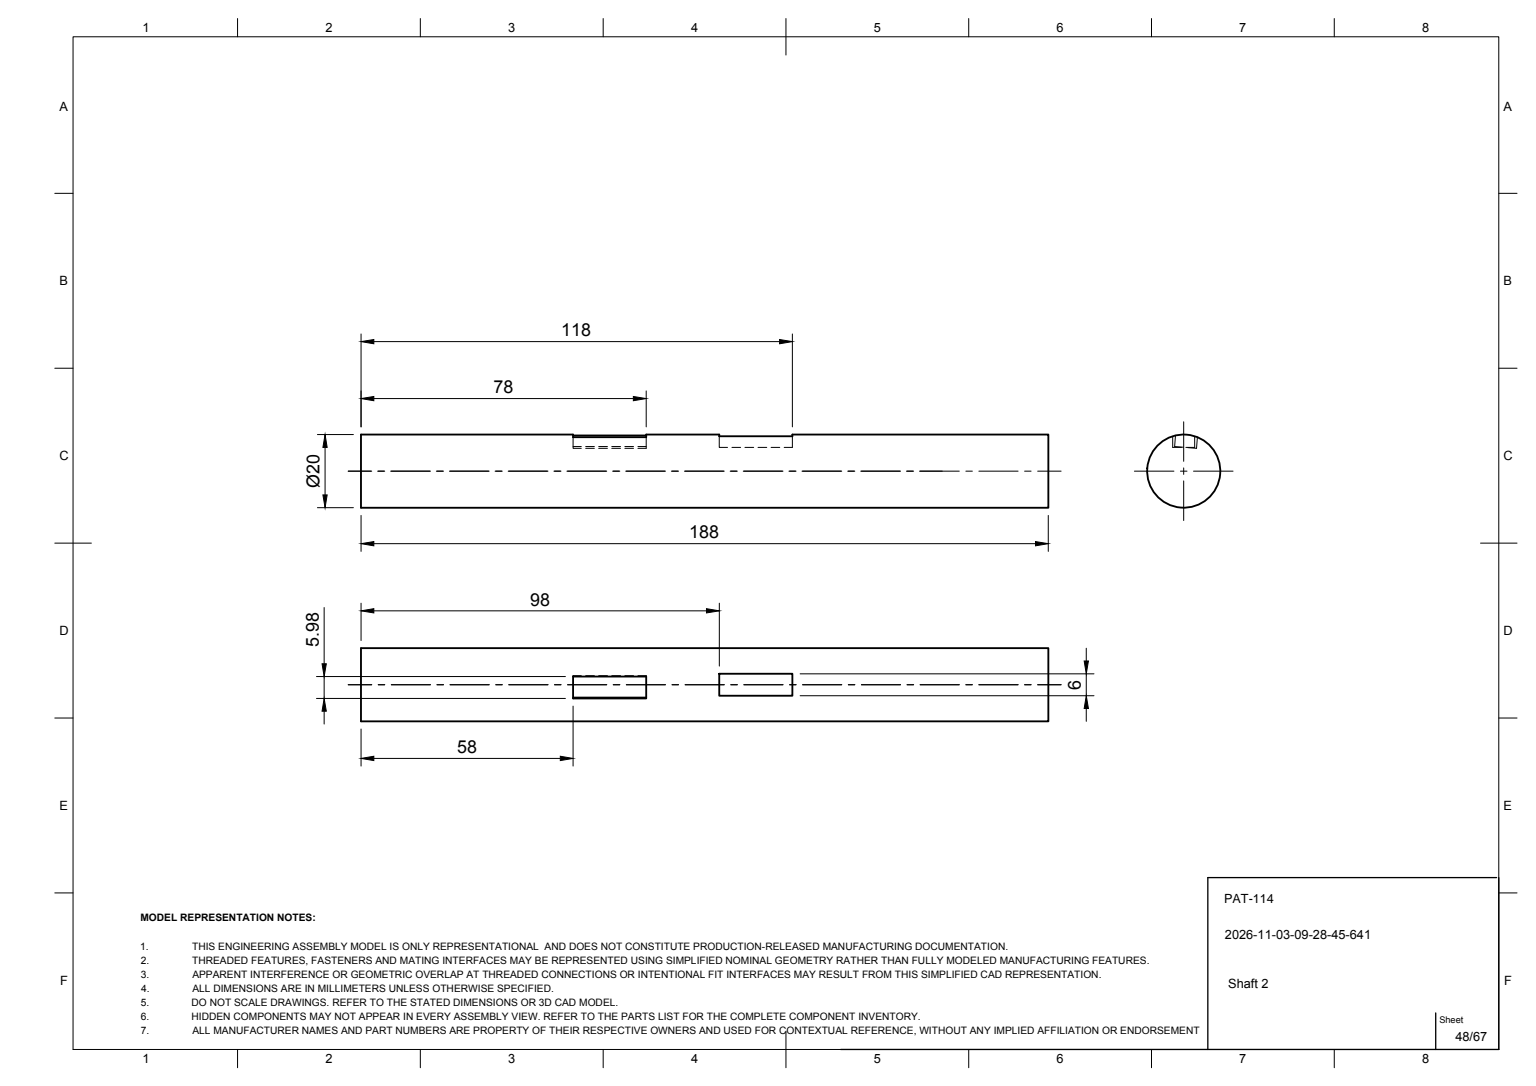
ISO-10303-21;
HEADER;
/* Generated by software containing ST-Developer
 * from STEP Tools, Inc. (www.steptools.com) 
 */

FILE_DESCRIPTION(
/* description */ ('Two-stage gear reducer in split housing'),
/* implementation_level */ '2;1');

FILE_NAME(
/* name */ 'Shaft 2.step',
/* time_stamp */ '2026-10-28T03:22:31-07:00',
/* author */ (''),
/* organization */ (''),
/* preprocessor_version */ 'ST-DEVELOPER v20.2',
/* originating_system */ 'Autodesk Translation Framework v15.17.0.0',
/* authorisation */ '');

FILE_SCHEMA (('AUTOMOTIVE_DESIGN { 1 0 10303 214 3 1 1 }'));
ENDSEC;

DATA;
#10=MECHANICAL_DESIGN_GEOMETRIC_PRESENTATION_REPRESENTATION('',(#1286),#73366);
#1159=SHAPE_REPRESENTATION_RELATIONSHIP('SRR','None',#73650,#1215);
#1215=ADVANCED_BREP_SHAPE_REPRESENTATION('',(#1355),#73346);
#1286=STYLED_ITEM('',(#73988),#1355);
#1355=MANIFOLD_SOLID_BREP('Body1',#16176);
#1558=FACE_BOUND('',#3660,.T.);
#1559=FACE_BOUND('',#3661,.T.);
#1858=PLANE('',#17950);
#1859=PLANE('',#17951);
#1860=PLANE('',#17953);
#1861=PLANE('',#17954);
#1862=PLANE('',#17955);
#1863=PLANE('',#17957);
#1864=PLANE('',#17958);
#1865=PLANE('',#17960);
#1866=PLANE('',#17961);
#1867=PLANE('',#17962);
#1868=PLANE('',#17967);
#1869=PLANE('',#17968);
#2552=FACE_OUTER_BOUND('',#3649,.T.);
#2553=FACE_OUTER_BOUND('',#3650,.T.);
#2554=FACE_OUTER_BOUND('',#3651,.T.);
#2555=FACE_OUTER_BOUND('',#3652,.T.);
#2556=FACE_OUTER_BOUND('',#3653,.T.);
#2557=FACE_OUTER_BOUND('',#3654,.T.);
#2558=FACE_OUTER_BOUND('',#3655,.T.);
#2559=FACE_OUTER_BOUND('',#3656,.T.);
#2560=FACE_OUTER_BOUND('',#3657,.T.);
#2561=FACE_OUTER_BOUND('',#3658,.T.);
#2562=FACE_OUTER_BOUND('',#3659,.T.);
#2563=FACE_OUTER_BOUND('',#3662,.T.);
#2564=FACE_OUTER_BOUND('',#3663,.T.);
#3649=EDGE_LOOP('',(#12989,#12990,#12991,#12992));
#3650=EDGE_LOOP('',(#12993,#12994,#12995,#12996));
#3651=EDGE_LOOP('',(#12997,#12998,#12999,#13000));
#3652=EDGE_LOOP('',(#13001,#13002,#13003,#13004));
#3653=EDGE_LOOP('',(#13005,#13006,#13007,#13008));
#3654=EDGE_LOOP('',(#13009,#13010,#13011,#13012));
#3655=EDGE_LOOP('',(#13013,#13014,#13015,#13016));
#3656=EDGE_LOOP('',(#13017,#13018,#13019,#13020));
#3657=EDGE_LOOP('',(#13021,#13022,#13023,#13024));
#3658=EDGE_LOOP('',(#13025,#13026,#13027,#13028));
#3659=EDGE_LOOP('',(#13029,#13030,#13031,#13032));
#3660=EDGE_LOOP('',(#13033,#13034,#13035,#13036));
#3661=EDGE_LOOP('',(#13037,#13038,#13039,#13040));
#3662=EDGE_LOOP('',(#13041));
#3663=EDGE_LOOP('',(#13042));
#4663=LINE('',#37341,#5687);
#4664=LINE('',#37343,#5688);
#4665=LINE('',#37345,#5689);
#4666=LINE('',#37346,#5690);
#4667=LINE('',#37351,#5691);
#4668=LINE('',#37352,#5692);
#4669=LINE('',#37355,#5693);
#4670=LINE('',#37357,#5694);
#4671=LINE('',#37358,#5695);
#4672=LINE('',#37360,#5696);
#4673=LINE('',#37366,#5697);
#4674=LINE('',#37368,#5698);
#4675=LINE('',#37370,#5699);
#4676=LINE('',#37371,#5700);
#4677=LINE('',#37376,#5701);
#4678=LINE('',#37377,#5702);
#4679=LINE('',#37380,#5703);
#4680=LINE('',#37382,#5704);
#4681=LINE('',#37383,#5705);
#4682=LINE('',#37385,#5706);
#4683=LINE('',#37392,#5707);
#5687=VECTOR('',#21343,1.);
#5688=VECTOR('',#21344,1.);
#5689=VECTOR('',#21345,1.);
#5690=VECTOR('',#21346,1.);
#5691=VECTOR('',#21351,1.);
#5692=VECTOR('',#21352,1.);
#5693=VECTOR('',#21355,1.);
#5694=VECTOR('',#21356,1.);
#5695=VECTOR('',#21357,1.);
#5696=VECTOR('',#21360,1.);
#5697=VECTOR('',#21367,1.);
#5698=VECTOR('',#21368,1.);
#5699=VECTOR('',#21369,1.);
#5700=VECTOR('',#21370,1.);
#5701=VECTOR('',#21375,1.);
#5702=VECTOR('',#21376,1.);
#5703=VECTOR('',#21379,1.);
#5704=VECTOR('',#21380,1.);
#5705=VECTOR('',#21381,1.);
#5706=VECTOR('',#21384,1.);
#5707=VECTOR('',#21393,1.);
#6618=CIRCLE('',#17952,1.);
#6619=CIRCLE('',#17956,1.);
#6620=CIRCLE('',#17959,1.);
#6621=CIRCLE('',#17963,1.);
#6622=CIRCLE('',#17965,1.);
#6623=CIRCLE('',#17966,1.);
#7667=VERTEX_POINT('',#37339);
#7668=VERTEX_POINT('',#37340);
#7669=VERTEX_POINT('',#37342);
#7670=VERTEX_POINT('',#37344);
#7671=VERTEX_POINT('',#37348);
#7672=VERTEX_POINT('',#37350);
#7673=VERTEX_POINT('',#37354);
#7674=VERTEX_POINT('',#37356);
#7675=VERTEX_POINT('',#37364);
#7676=VERTEX_POINT('',#37365);
#7677=VERTEX_POINT('',#37367);
#7678=VERTEX_POINT('',#37369);
#7679=VERTEX_POINT('',#37373);
#7680=VERTEX_POINT('',#37375);
#7681=VERTEX_POINT('',#37379);
#7682=VERTEX_POINT('',#37381);
#7683=VERTEX_POINT('',#37389);
#7684=VERTEX_POINT('',#37391);
#9548=EDGE_CURVE('',#7667,#7668,#4663,.T.);
#9549=EDGE_CURVE('',#7667,#7669,#4664,.T.);
#9550=EDGE_CURVE('',#7670,#7669,#4665,.T.);
#9551=EDGE_CURVE('',#7670,#7668,#4666,.T.);
#9552=EDGE_CURVE('',#7668,#7671,#6618,.T.);
#9553=EDGE_CURVE('',#7672,#7670,#4667,.T.);
#9554=EDGE_CURVE('',#7671,#7672,#4668,.T.);
#9555=EDGE_CURVE('',#7671,#7673,#4669,.T.);
#9556=EDGE_CURVE('',#7672,#7674,#4670,.T.);
#9557=EDGE_CURVE('',#7674,#7673,#4671,.T.);
#9558=EDGE_CURVE('',#7669,#7674,#4672,.T.);
#9559=EDGE_CURVE('',#7673,#7667,#6619,.T.);
#9560=EDGE_CURVE('',#7675,#7676,#4673,.T.);
#9561=EDGE_CURVE('',#7675,#7677,#4674,.T.);
#9562=EDGE_CURVE('',#7678,#7677,#4675,.T.);
#9563=EDGE_CURVE('',#7678,#7676,#4676,.T.);
#9564=EDGE_CURVE('',#7676,#7679,#6620,.T.);
#9565=EDGE_CURVE('',#7680,#7678,#4677,.T.);
#9566=EDGE_CURVE('',#7679,#7680,#4678,.T.);
#9567=EDGE_CURVE('',#7679,#7681,#4679,.T.);
#9568=EDGE_CURVE('',#7680,#7682,#4680,.T.);
#9569=EDGE_CURVE('',#7682,#7681,#4681,.T.);
#9570=EDGE_CURVE('',#7677,#7682,#4682,.T.);
#9571=EDGE_CURVE('',#7681,#7675,#6621,.T.);
#9572=EDGE_CURVE('',#7683,#7683,#6622,.T.);
#9573=EDGE_CURVE('',#7683,#7684,#4683,.T.);
#9574=EDGE_CURVE('',#7684,#7684,#6623,.T.);
#12989=ORIENTED_EDGE('',*,*,#9548,.F.);
#12990=ORIENTED_EDGE('',*,*,#9549,.T.);
#12991=ORIENTED_EDGE('',*,*,#9550,.F.);
#12992=ORIENTED_EDGE('',*,*,#9551,.T.);
#12993=ORIENTED_EDGE('',*,*,#9552,.F.);
#12994=ORIENTED_EDGE('',*,*,#9551,.F.);
#12995=ORIENTED_EDGE('',*,*,#9553,.F.);
#12996=ORIENTED_EDGE('',*,*,#9554,.F.);
#12997=ORIENTED_EDGE('',*,*,#9555,.F.);
#12998=ORIENTED_EDGE('',*,*,#9554,.T.);
#12999=ORIENTED_EDGE('',*,*,#9556,.T.);
#13000=ORIENTED_EDGE('',*,*,#9557,.T.);
#13001=ORIENTED_EDGE('',*,*,#9553,.T.);
#13002=ORIENTED_EDGE('',*,*,#9550,.T.);
#13003=ORIENTED_EDGE('',*,*,#9558,.T.);
#13004=ORIENTED_EDGE('',*,*,#9556,.F.);
#13005=ORIENTED_EDGE('',*,*,#9559,.F.);
#13006=ORIENTED_EDGE('',*,*,#9557,.F.);
#13007=ORIENTED_EDGE('',*,*,#9558,.F.);
#13008=ORIENTED_EDGE('',*,*,#9549,.F.);
#13009=ORIENTED_EDGE('',*,*,#9560,.F.);
#13010=ORIENTED_EDGE('',*,*,#9561,.T.);
#13011=ORIENTED_EDGE('',*,*,#9562,.F.);
#13012=ORIENTED_EDGE('',*,*,#9563,.T.);
#13013=ORIENTED_EDGE('',*,*,#9564,.F.);
#13014=ORIENTED_EDGE('',*,*,#9563,.F.);
#13015=ORIENTED_EDGE('',*,*,#9565,.F.);
#13016=ORIENTED_EDGE('',*,*,#9566,.F.);
#13017=ORIENTED_EDGE('',*,*,#9567,.F.);
#13018=ORIENTED_EDGE('',*,*,#9566,.T.);
#13019=ORIENTED_EDGE('',*,*,#9568,.T.);
#13020=ORIENTED_EDGE('',*,*,#9569,.T.);
#13021=ORIENTED_EDGE('',*,*,#9565,.T.);
#13022=ORIENTED_EDGE('',*,*,#9562,.T.);
#13023=ORIENTED_EDGE('',*,*,#9570,.T.);
#13024=ORIENTED_EDGE('',*,*,#9568,.F.);
#13025=ORIENTED_EDGE('',*,*,#9571,.F.);
#13026=ORIENTED_EDGE('',*,*,#9569,.F.);
#13027=ORIENTED_EDGE('',*,*,#9570,.F.);
#13028=ORIENTED_EDGE('',*,*,#9561,.F.);
#13029=ORIENTED_EDGE('',*,*,#9572,.F.);
#13030=ORIENTED_EDGE('',*,*,#9573,.T.);
#13031=ORIENTED_EDGE('',*,*,#9574,.T.);
#13032=ORIENTED_EDGE('',*,*,#9573,.F.);
#13033=ORIENTED_EDGE('',*,*,#9555,.T.);
#13034=ORIENTED_EDGE('',*,*,#9559,.T.);
#13035=ORIENTED_EDGE('',*,*,#9548,.T.);
#13036=ORIENTED_EDGE('',*,*,#9552,.T.);
#13037=ORIENTED_EDGE('',*,*,#9567,.T.);
#13038=ORIENTED_EDGE('',*,*,#9571,.T.);
#13039=ORIENTED_EDGE('',*,*,#9560,.T.);
#13040=ORIENTED_EDGE('',*,*,#9564,.T.);
#13041=ORIENTED_EDGE('',*,*,#9572,.T.);
#13042=ORIENTED_EDGE('',*,*,#9574,.F.);
#15112=CYLINDRICAL_SURFACE('',#17964,1.);
#15759=ADVANCED_FACE('',(#2552),#1858,.F.);
#15760=ADVANCED_FACE('',(#2553),#1859,.T.);
#15761=ADVANCED_FACE('',(#2554),#1860,.F.);
#15762=ADVANCED_FACE('',(#2555),#1861,.F.);
#15763=ADVANCED_FACE('',(#2556),#1862,.F.);
#15764=ADVANCED_FACE('',(#2557),#1863,.F.);
#15765=ADVANCED_FACE('',(#2558),#1864,.T.);
#15766=ADVANCED_FACE('',(#2559),#1865,.F.);
#15767=ADVANCED_FACE('',(#2560),#1866,.F.);
#15768=ADVANCED_FACE('',(#2561),#1867,.F.);
#15769=ADVANCED_FACE('',(#2562,#1558,#1559),#15112,.T.);
#15770=ADVANCED_FACE('',(#2563),#1868,.T.);
#15771=ADVANCED_FACE('',(#2564),#1869,.F.);
#16176=CLOSED_SHELL('',(#15759,#15760,#15761,#15762,#15763,#15764,#15765,
#15766,#15767,#15768,#15769,#15770,#15771));
#17949=AXIS2_PLACEMENT_3D('',#37337,#21339,#21340);
#17950=AXIS2_PLACEMENT_3D('',#37338,#21341,#21342);
#17951=AXIS2_PLACEMENT_3D('',#37347,#21347,#21348);
#17952=AXIS2_PLACEMENT_3D('',#37349,#21349,#21350);
#17953=AXIS2_PLACEMENT_3D('',#37353,#21353,#21354);
#17954=AXIS2_PLACEMENT_3D('',#37359,#21358,#21359);
#17955=AXIS2_PLACEMENT_3D('',#37361,#21361,#21362);
#17956=AXIS2_PLACEMENT_3D('',#37362,#21363,#21364);
#17957=AXIS2_PLACEMENT_3D('',#37363,#21365,#21366);
#17958=AXIS2_PLACEMENT_3D('',#37372,#21371,#21372);
#17959=AXIS2_PLACEMENT_3D('',#37374,#21373,#21374);
#17960=AXIS2_PLACEMENT_3D('',#37378,#21377,#21378);
#17961=AXIS2_PLACEMENT_3D('',#37384,#21382,#21383);
#17962=AXIS2_PLACEMENT_3D('',#37386,#21385,#21386);
#17963=AXIS2_PLACEMENT_3D('',#37387,#21387,#21388);
#17964=AXIS2_PLACEMENT_3D('',#37388,#21389,#21390);
#17965=AXIS2_PLACEMENT_3D('',#37390,#21391,#21392);
#17966=AXIS2_PLACEMENT_3D('',#37393,#21394,#21395);
#17967=AXIS2_PLACEMENT_3D('',#37394,#21396,#21397);
#17968=AXIS2_PLACEMENT_3D('',#37395,#21398,#21399);
#21339=DIRECTION('axis',(0.,0.,1.));
#21340=DIRECTION('refdir',(1.,0.,0.));
#21341=DIRECTION('center_axis',(-1.,0.,0.));
#21342=DIRECTION('ref_axis',(0.,0.,1.));
#21343=DIRECTION('',(0.,-1.,0.));
#21344=DIRECTION('',(0.,0.,1.));
#21345=DIRECTION('',(0.,1.,0.));
#21346=DIRECTION('',(0.,0.,-1.));
#21347=DIRECTION('center_axis',(0.,1.,0.));
#21348=DIRECTION('ref_axis',(1.,0.,0.));
#21349=DIRECTION('center_axis',(0.,-1.,0.));
#21350=DIRECTION('ref_axis',(1.,0.,0.));
#21351=DIRECTION('',(-1.,0.,0.));
#21352=DIRECTION('',(0.,0.,1.));
#21353=DIRECTION('center_axis',(1.,0.,0.));
#21354=DIRECTION('ref_axis',(0.,0.,-1.));
#21355=DIRECTION('',(0.,1.,0.));
#21356=DIRECTION('',(0.,1.,0.));
#21357=DIRECTION('',(0.,0.,-1.));
#21358=DIRECTION('center_axis',(0.,0.,1.));
#21359=DIRECTION('ref_axis',(1.,0.,0.));
#21360=DIRECTION('',(1.,0.,0.));
#21361=DIRECTION('center_axis',(0.,1.,0.));
#21362=DIRECTION('ref_axis',(0.,0.,1.));
#21363=DIRECTION('center_axis',(0.,1.,0.));
#21364=DIRECTION('ref_axis',(1.,0.,0.));
#21365=DIRECTION('center_axis',(-0.996917333733128,0.,0.0784590957278455));
#21366=DIRECTION('ref_axis',(0.0784590957278455,0.,0.996917333733128));
#21367=DIRECTION('',(0.,-1.,0.));
#21368=DIRECTION('',(0.0784590957278455,0.,0.996917333733128));
#21369=DIRECTION('',(0.,1.,0.));
#21370=DIRECTION('',(-0.0784590957278455,0.,-0.996917333733128));
#21371=DIRECTION('center_axis',(0.,1.,0.));
#21372=DIRECTION('ref_axis',(1.,0.,0.));
#21373=DIRECTION('center_axis',(0.,-1.,0.));
#21374=DIRECTION('ref_axis',(1.,0.,0.));
#21375=DIRECTION('',(-0.996917333733128,0.,0.0784590957278475));
#21376=DIRECTION('',(0.0784590957278456,0.,0.996917333733128));
#21377=DIRECTION('center_axis',(0.996917333733128,0.,-0.0784590957278456));
#21378=DIRECTION('ref_axis',(-0.0784590957278456,0.,-0.996917333733128));
#21379=DIRECTION('',(0.,1.,0.));
#21380=DIRECTION('',(0.,1.,0.));
#21381=DIRECTION('',(-0.0784590957278456,0.,-0.996917333733128));
#21382=DIRECTION('center_axis',(0.0784590957278475,0.,0.996917333733128));
#21383=DIRECTION('ref_axis',(0.996917333733128,0.,-0.0784590957278475));
#21384=DIRECTION('',(0.996917333733128,0.,-0.0784590957278475));
#21385=DIRECTION('center_axis',(0.,1.,0.));
#21386=DIRECTION('ref_axis',(0.,0.,1.));
#21387=DIRECTION('center_axis',(0.,1.,0.));
#21388=DIRECTION('ref_axis',(1.,0.,0.));
#21389=DIRECTION('center_axis',(0.,1.,0.));
#21390=DIRECTION('ref_axis',(1.,0.,0.));
#21391=DIRECTION('center_axis',(0.,1.,0.));
#21392=DIRECTION('ref_axis',(1.,0.,0.));
#21393=DIRECTION('',(0.,-1.,0.));
#21394=DIRECTION('center_axis',(0.,1.,0.));
#21395=DIRECTION('ref_axis',(1.,0.,0.));
#21396=DIRECTION('center_axis',(0.,1.,0.));
#21397=DIRECTION('ref_axis',(1.,0.,0.));
#21398=DIRECTION('center_axis',(0.,1.,0.));
#21399=DIRECTION('ref_axis',(1.,0.,0.));
#37337=CARTESIAN_POINT('',(0.,0.,0.));
#37338=CARTESIAN_POINT('Origin',(5.7,1.6,8.));
#37339=CARTESIAN_POINT('',(5.7,3.6,9.04606079858305));
#37340=CARTESIAN_POINT('',(5.7,1.6,9.04606079858305));
#37341=CARTESIAN_POINT('',(5.7,-9.4,9.04606079858305));
#37342=CARTESIAN_POINT('',(5.7,3.6,9.35));
#37343=CARTESIAN_POINT('',(5.7,3.6,9.35));
#37344=CARTESIAN_POINT('',(5.7,1.6,9.35));
#37345=CARTESIAN_POINT('',(5.7,1.6,9.35));
#37346=CARTESIAN_POINT('',(5.7,1.6,9.35));
#37347=CARTESIAN_POINT('Origin',(6.,1.6,8.675));
#37348=CARTESIAN_POINT('',(6.3,1.6,9.04606079858305));
#37349=CARTESIAN_POINT('Origin',(6.,1.6,10.));
#37350=CARTESIAN_POINT('',(6.3,1.6,9.35));
#37351=CARTESIAN_POINT('',(6.3,1.6,9.35));
#37352=CARTESIAN_POINT('',(6.3,1.6,8.));
#37353=CARTESIAN_POINT('Origin',(6.3,1.6,9.35));
#37354=CARTESIAN_POINT('',(6.3,3.6,9.04606079858305));
#37355=CARTESIAN_POINT('',(6.3,-9.4,9.04606079858305));
#37356=CARTESIAN_POINT('',(6.3,3.6,9.35));
#37357=CARTESIAN_POINT('',(6.3,1.6,9.35));
#37358=CARTESIAN_POINT('',(6.3,3.6,8.));
#37359=CARTESIAN_POINT('Origin',(5.7,1.6,9.35));
#37360=CARTESIAN_POINT('',(6.3,3.6,9.35));
#37361=CARTESIAN_POINT('Origin',(6.,3.6,8.675));
#37362=CARTESIAN_POINT('Origin',(6.,3.6,10.));
#37363=CARTESIAN_POINT('Origin',(5.54400660842437,-2.4,8.0297030612521));
#37364=CARTESIAN_POINT('',(5.62607959275755,-0.4,9.07253920349826));
#37365=CARTESIAN_POINT('',(5.62607959275755,-2.4,9.07253920349826));
#37366=CARTESIAN_POINT('',(5.62607959275755,-9.4,9.07253920349826));
#37367=CARTESIAN_POINT('',(5.64992638765696,-0.4,9.37554146179182));
#37368=CARTESIAN_POINT('',(5.64992638765696,-0.4,9.37554146179182));
#37369=CARTESIAN_POINT('',(5.64992638765696,-2.4,9.37554146179182));
#37370=CARTESIAN_POINT('',(5.64992638765696,-2.4,9.37554146179182));
#37371=CARTESIAN_POINT('',(5.64992638765696,-2.4,9.37554146179182));
#37372=CARTESIAN_POINT('Origin',(5.89604169816061,-2.4,8.67908453280361));
#37373=CARTESIAN_POINT('',(6.22422999299742,-2.4,9.02546374606156));
#37374=CARTESIAN_POINT('Origin',(6.,-2.4,10.));
#37375=CARTESIAN_POINT('',(6.24807678789684,-2.4,9.32846600435511));
#37376=CARTESIAN_POINT('',(6.24807678789684,-2.4,9.32846600435511));
#37377=CARTESIAN_POINT('',(6.14215700866425,-2.4,7.98262760381539));
#37378=CARTESIAN_POINT('Origin',(6.24807678789684,-2.4,9.32846600435511));
#37379=CARTESIAN_POINT('',(6.22422999299742,-0.4,9.02546374606156));
#37380=CARTESIAN_POINT('',(6.22422999299742,-9.4,9.02546374606156));
#37381=CARTESIAN_POINT('',(6.24807678789684,-0.4,9.32846600435511));
#37382=CARTESIAN_POINT('',(6.24807678789684,-2.4,9.32846600435511));
#37383=CARTESIAN_POINT('',(6.14215700866425,-0.4,7.98262760381539));
#37384=CARTESIAN_POINT('Origin',(5.64992638765696,-2.4,9.37554146179182));
#37385=CARTESIAN_POINT('',(6.24807678789684,-0.4,9.32846600435511));
#37386=CARTESIAN_POINT('Origin',(5.89604169816061,-0.4,8.67908453280361));
#37387=CARTESIAN_POINT('Origin',(6.,-0.4,10.));
#37388=CARTESIAN_POINT('Origin',(6.,-9.4,10.));
#37389=CARTESIAN_POINT('',(5.,9.4,10.));
#37390=CARTESIAN_POINT('Origin',(6.,9.4,10.));
#37391=CARTESIAN_POINT('',(5.,-9.4,10.));
#37392=CARTESIAN_POINT('',(5.,-9.4,10.));
#37393=CARTESIAN_POINT('Origin',(6.,-9.4,10.));
#37394=CARTESIAN_POINT('Origin',(6.,9.4,10.));
#37395=CARTESIAN_POINT('Origin',(6.,-9.4,10.));
#73282=UNCERTAINTY_MEASURE_WITH_UNIT(LENGTH_MEASURE(0.001),#73367,
'DISTANCE_ACCURACY_VALUE',
'Maximum model space distance between geometric entities at asserted c
onnectivities');
#73302=UNCERTAINTY_MEASURE_WITH_UNIT(LENGTH_MEASURE(0.001),#73367,
'DISTANCE_ACCURACY_VALUE',
'Maximum model space distance between geometric entities at asserted c
onnectivities');
#73346=(
GEOMETRIC_REPRESENTATION_CONTEXT(3)
GLOBAL_UNCERTAINTY_ASSIGNED_CONTEXT((#73282))
GLOBAL_UNIT_ASSIGNED_CONTEXT((#73367,#73369,#73370))
REPRESENTATION_CONTEXT('','3D')
);
#73366=(
GEOMETRIC_REPRESENTATION_CONTEXT(3)
GLOBAL_UNCERTAINTY_ASSIGNED_CONTEXT((#73302))
GLOBAL_UNIT_ASSIGNED_CONTEXT((#73367,#73369,#73370))
REPRESENTATION_CONTEXT('','3D')
);
#73367=(
LENGTH_UNIT()
NAMED_UNIT(*)
SI_UNIT(.CENTI.,.METRE.)
);
#73369=(
NAMED_UNIT(*)
PLANE_ANGLE_UNIT()
SI_UNIT($,.RADIAN.)
);
#73370=(
NAMED_UNIT(*)
SI_UNIT($,.STERADIAN.)
SOLID_ANGLE_UNIT()
);
#73414=SHAPE_DEFINITION_REPRESENTATION(#73547,#73650);
#73547=PRODUCT_DEFINITION_SHAPE('',$,#73714);
#73650=SHAPE_REPRESENTATION('',(#17949),#73346);
#73670=PRODUCT_DEFINITION_CONTEXT('part definition',#73861,'design');
#73714=PRODUCT_DEFINITION('Shaft 2','Shaft 2',#73777,#73670);
#73777=PRODUCT_DEFINITION_FORMATION('',$,#73906);
#73861=APPLICATION_CONTEXT(
'Core Data for Automotive Mechanical Design Process');
#73862=PRODUCT_CONTEXT('part definition',#73861,'mechanical');
#73906=PRODUCT('Shaft 2','Shaft 2','Shaft 2',(#73862));
#73982=COLOUR_RGB('Grey',0.48,0.52,0.57);
#73983=FILL_AREA_STYLE_COLOUR('',#73982);
#73984=FILL_AREA_STYLE('',(#73983));
#73985=SURFACE_STYLE_FILL_AREA(#73984);
#73986=SURFACE_SIDE_STYLE('',(#73985));
#73987=SURFACE_STYLE_USAGE(.BOTH.,#73986);
#73988=PRESENTATION_STYLE_ASSIGNMENT((#73987));
ENDSEC;
END-ISO-10303-21;
